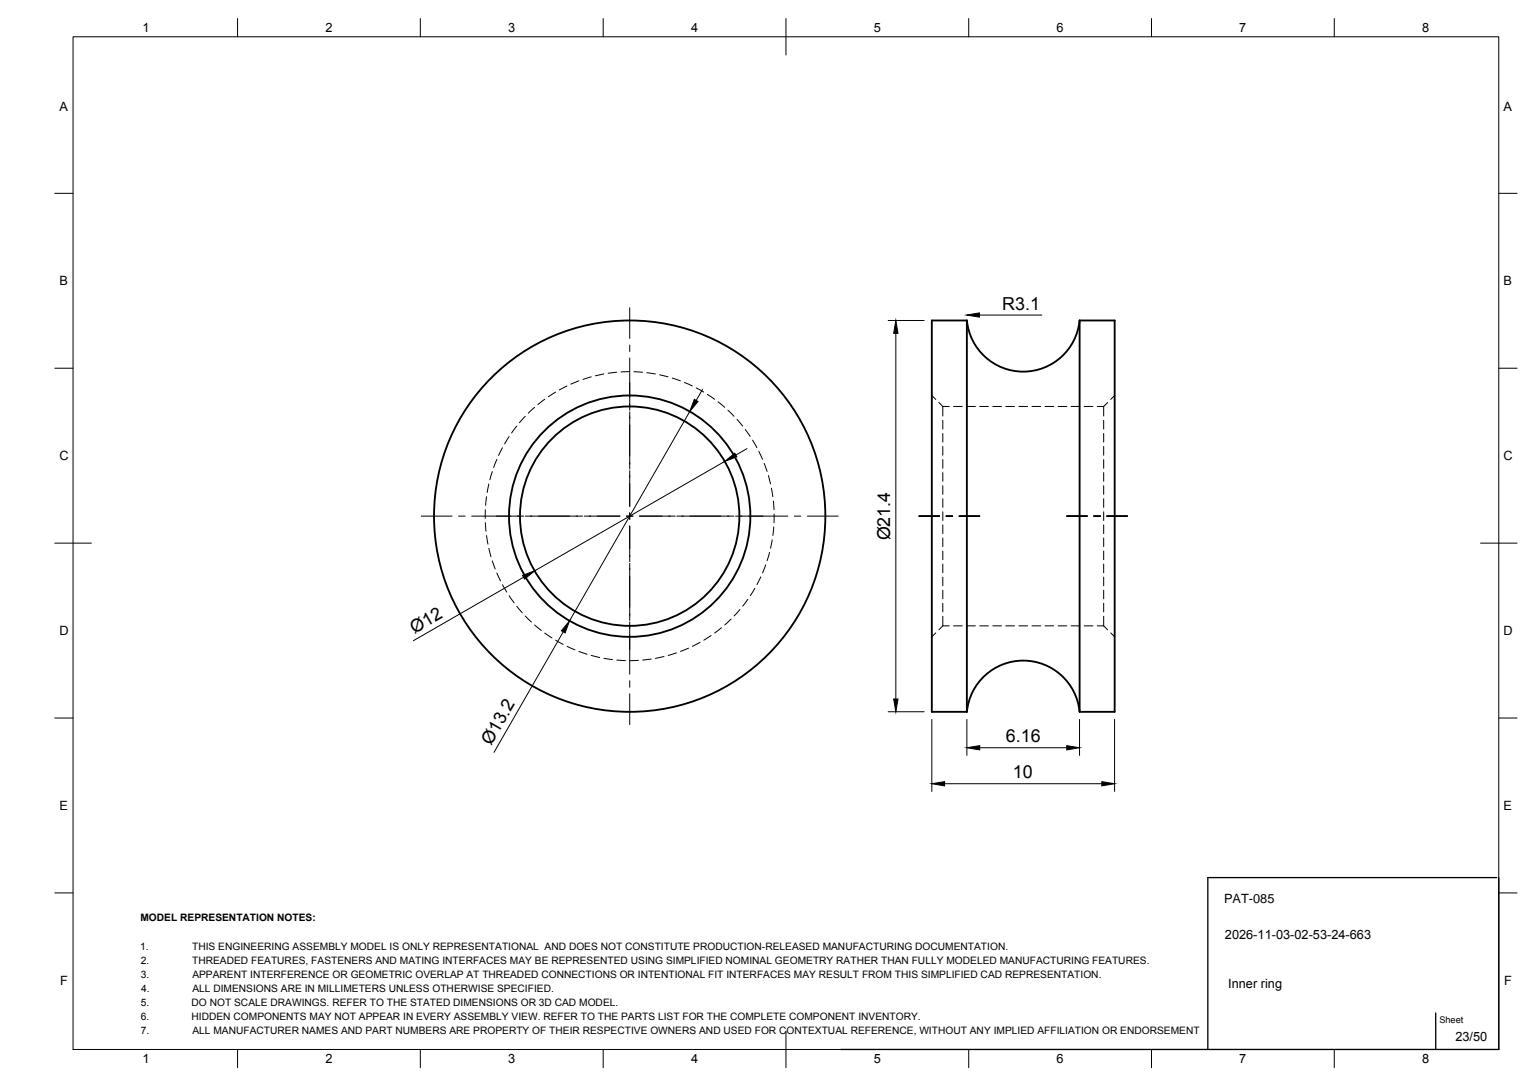
ISO-10303-21;
HEADER;
/* Generated by software containing ST-Developer
 * from STEP Tools, Inc. (www.steptools.com) 
 */

FILE_DESCRIPTION(
/* description */ ('Rack and pinion manual slide'),
/* implementation_level */ '2;1');

FILE_NAME(
/* name */ 'Inner ring.step',
/* time_stamp */ '2026-10-28T03:22:49-07:00',
/* author */ (''),
/* organization */ (''),
/* preprocessor_version */ 'ST-DEVELOPER v20.2',
/* originating_system */ 'Autodesk Translation Framework v15.17.0.0',
/* authorisation */ '');

FILE_SCHEMA (('AUTOMOTIVE_DESIGN { 1 0 10303 214 3 1 1 }'));
ENDSEC;

DATA;
#10=MECHANICAL_DESIGN_GEOMETRIC_PRESENTATION_REPRESENTATION('',(#751),#34851);
#603=TOROIDAL_SURFACE('',#14780,1.1,0.309556);
#620=CONICAL_SURFACE('',#14791,0.63,0.785398163397448);
#621=CONICAL_SURFACE('',#14798,0.63,0.785398163397448);
#659=SHAPE_REPRESENTATION_RELATIONSHIP('SRR','None',#35095,#705);
#705=ADVANCED_BREP_SHAPE_REPRESENTATION('',(#803),#34820);
#751=STYLED_ITEM('',(#35411),#803);
#803=MANIFOLD_SOLID_BREP('Body1',#13772);
#975=FACE_BOUND('',#2684,.T.);
#976=FACE_BOUND('',#2687,.T.);
#1218=PLANE('',#14793);
#1219=PLANE('',#14796);
#1798=FACE_OUTER_BOUND('',#2679,.T.);
#1799=FACE_OUTER_BOUND('',#2680,.T.);
#1800=FACE_OUTER_BOUND('',#2681,.T.);
#1801=FACE_OUTER_BOUND('',#2682,.T.);
#1802=FACE_OUTER_BOUND('',#2683,.T.);
#1803=FACE_OUTER_BOUND('',#2685,.T.);
#1804=FACE_OUTER_BOUND('',#2686,.T.);
#1805=FACE_OUTER_BOUND('',#2688,.T.);
#2679=EDGE_LOOP('',(#10490,#10491,#10492,#10493,#10494,#10495));
#2680=EDGE_LOOP('',(#10496,#10497,#10498,#10499,#10500));
#2681=EDGE_LOOP('',(#10501,#10502,#10503,#10504));
#2682=EDGE_LOOP('',(#10505,#10506,#10507,#10508));
#2683=EDGE_LOOP('',(#10509));
#2684=EDGE_LOOP('',(#10510));
#2685=EDGE_LOOP('',(#10511,#10512,#10513,#10514,#10515));
#2686=EDGE_LOOP('',(#10516));
#2687=EDGE_LOOP('',(#10517));
#2688=EDGE_LOOP('',(#10518,#10519,#10520,#10521));
#3675=LINE('',#20800,#4966);
#3676=LINE('',#20806,#4967);
#3677=LINE('',#20810,#4968);
#3678=LINE('',#20816,#4969);
#3679=LINE('',#20821,#4970);
#4966=VECTOR('',#16991,1.070235);
#4967=VECTOR('',#16998,0.6);
#4968=VECTOR('',#17003,0.63);
#4969=VECTOR('',#17012,1.070235);
#4970=VECTOR('',#17019,0.63);
#5981=CIRCLE('',#14781,1.070235);
#5982=CIRCLE('',#14782,1.070235);
#5983=CIRCLE('',#14783,0.309556);
#5984=CIRCLE('',#14784,1.070235);
#5985=CIRCLE('',#14785,1.070235);
#5986=CIRCLE('',#14787,1.070235);
#5987=CIRCLE('',#14789,0.6);
#5988=CIRCLE('',#14790,0.6);
#5989=CIRCLE('',#14792,0.66);
#5990=CIRCLE('',#14795,1.070235);
#5991=CIRCLE('',#14797,0.66);
#6641=VERTEX_POINT('',#20789);
#6642=VERTEX_POINT('',#20790);
#6643=VERTEX_POINT('',#20793);
#6644=VERTEX_POINT('',#20795);
#6645=VERTEX_POINT('',#20799);
#6646=VERTEX_POINT('',#20803);
#6647=VERTEX_POINT('',#20805);
#6648=VERTEX_POINT('',#20809);
#6649=VERTEX_POINT('',#20814);
#6650=VERTEX_POINT('',#20818);
#8057=EDGE_CURVE('',#6641,#6642,#5981,.T.);
#8058=EDGE_CURVE('',#6642,#6641,#5982,.T.);
#8059=EDGE_CURVE('',#6642,#6643,#5983,.T.);
#8060=EDGE_CURVE('',#6644,#6643,#5984,.T.);
#8061=EDGE_CURVE('',#6643,#6644,#5985,.T.);
#8062=EDGE_CURVE('',#6644,#6645,#3675,.T.);
#8063=EDGE_CURVE('',#6645,#6645,#5986,.T.);
#8064=EDGE_CURVE('',#6646,#6646,#5987,.T.);
#8065=EDGE_CURVE('',#6646,#6647,#3676,.T.);
#8066=EDGE_CURVE('',#6647,#6647,#5988,.T.);
#8067=EDGE_CURVE('',#6647,#6648,#3677,.T.);
#8068=EDGE_CURVE('',#6648,#6648,#5989,.T.);
#8069=EDGE_CURVE('',#6649,#6649,#5990,.T.);
#8070=EDGE_CURVE('',#6649,#6641,#3678,.T.);
#8071=EDGE_CURVE('',#6650,#6650,#5991,.T.);
#8072=EDGE_CURVE('',#6650,#6646,#3679,.T.);
#10490=ORIENTED_EDGE('',*,*,#8057,.F.);
#10491=ORIENTED_EDGE('',*,*,#8058,.F.);
#10492=ORIENTED_EDGE('',*,*,#8059,.T.);
#10493=ORIENTED_EDGE('',*,*,#8060,.F.);
#10494=ORIENTED_EDGE('',*,*,#8061,.F.);
#10495=ORIENTED_EDGE('',*,*,#8059,.F.);
#10496=ORIENTED_EDGE('',*,*,#8060,.T.);
#10497=ORIENTED_EDGE('',*,*,#8061,.T.);
#10498=ORIENTED_EDGE('',*,*,#8062,.T.);
#10499=ORIENTED_EDGE('',*,*,#8063,.T.);
#10500=ORIENTED_EDGE('',*,*,#8062,.F.);
#10501=ORIENTED_EDGE('',*,*,#8064,.T.);
#10502=ORIENTED_EDGE('',*,*,#8065,.T.);
#10503=ORIENTED_EDGE('',*,*,#8066,.F.);
#10504=ORIENTED_EDGE('',*,*,#8065,.F.);
#10505=ORIENTED_EDGE('',*,*,#8066,.T.);
#10506=ORIENTED_EDGE('',*,*,#8067,.T.);
#10507=ORIENTED_EDGE('',*,*,#8068,.F.);
#10508=ORIENTED_EDGE('',*,*,#8067,.F.);
#10509=ORIENTED_EDGE('',*,*,#8063,.F.);
#10510=ORIENTED_EDGE('',*,*,#8068,.T.);
#10511=ORIENTED_EDGE('',*,*,#8069,.F.);
#10512=ORIENTED_EDGE('',*,*,#8070,.T.);
#10513=ORIENTED_EDGE('',*,*,#8057,.T.);
#10514=ORIENTED_EDGE('',*,*,#8058,.T.);
#10515=ORIENTED_EDGE('',*,*,#8070,.F.);
#10516=ORIENTED_EDGE('',*,*,#8069,.T.);
#10517=ORIENTED_EDGE('',*,*,#8071,.F.);
#10518=ORIENTED_EDGE('',*,*,#8071,.T.);
#10519=ORIENTED_EDGE('',*,*,#8072,.T.);
#10520=ORIENTED_EDGE('',*,*,#8064,.F.);
#10521=ORIENTED_EDGE('',*,*,#8072,.F.);
#12928=CYLINDRICAL_SURFACE('',#14786,1.070235);
#12929=CYLINDRICAL_SURFACE('',#14788,0.6);
#12930=CYLINDRICAL_SURFACE('',#14794,1.070235);
#13276=ADVANCED_FACE('',(#1798),#603,.F.);
#13277=ADVANCED_FACE('',(#1799),#12928,.T.);
#13278=ADVANCED_FACE('',(#1800),#12929,.F.);
#13279=ADVANCED_FACE('',(#1801),#620,.F.);
#13280=ADVANCED_FACE('',(#1802,#975),#1218,.T.);
#13281=ADVANCED_FACE('',(#1803),#12930,.T.);
#13282=ADVANCED_FACE('',(#1804,#976),#1219,.T.);
#13283=ADVANCED_FACE('',(#1805),#621,.F.);
#13772=CLOSED_SHELL('',(#13276,#13277,#13278,#13279,#13280,#13281,#13282,
#13283));
#14779=AXIS2_PLACEMENT_3D('',#20787,#16975,#16976);
#14780=AXIS2_PLACEMENT_3D('',#20788,#16977,#16978);
#14781=AXIS2_PLACEMENT_3D('',#20791,#16979,#16980);
#14782=AXIS2_PLACEMENT_3D('',#20792,#16981,#16982);
#14783=AXIS2_PLACEMENT_3D('',#20794,#16983,#16984);
#14784=AXIS2_PLACEMENT_3D('',#20796,#16985,#16986);
#14785=AXIS2_PLACEMENT_3D('',#20797,#16987,#16988);
#14786=AXIS2_PLACEMENT_3D('',#20798,#16989,#16990);
#14787=AXIS2_PLACEMENT_3D('',#20801,#16992,#16993);
#14788=AXIS2_PLACEMENT_3D('',#20802,#16994,#16995);
#14789=AXIS2_PLACEMENT_3D('',#20804,#16996,#16997);
#14790=AXIS2_PLACEMENT_3D('',#20807,#16999,#17000);
#14791=AXIS2_PLACEMENT_3D('',#20808,#17001,#17002);
#14792=AXIS2_PLACEMENT_3D('',#20811,#17004,#17005);
#14793=AXIS2_PLACEMENT_3D('',#20812,#17006,#17007);
#14794=AXIS2_PLACEMENT_3D('',#20813,#17008,#17009);
#14795=AXIS2_PLACEMENT_3D('',#20815,#17010,#17011);
#14796=AXIS2_PLACEMENT_3D('',#20817,#17013,#17014);
#14797=AXIS2_PLACEMENT_3D('',#20819,#17015,#17016);
#14798=AXIS2_PLACEMENT_3D('',#20820,#17017,#17018);
#16975=DIRECTION('axis',(0.,0.,1.));
#16976=DIRECTION('refdir',(1.,0.,0.));
#16977=DIRECTION('center_axis',(0.,-1.,0.));
#16978=DIRECTION('ref_axis',(0.,0.,-1.));
#16979=DIRECTION('center_axis',(0.,-1.,0.));
#16980=DIRECTION('ref_axis',(1.,0.,0.));
#16981=DIRECTION('center_axis',(0.,-1.,0.));
#16982=DIRECTION('ref_axis',(1.,0.,0.));
#16983=DIRECTION('center_axis',(1.,0.,1.22464679914735E-16));
#16984=DIRECTION('ref_axis',(-1.22464679914735E-16,0.,1.));
#16985=DIRECTION('center_axis',(0.,1.,0.));
#16986=DIRECTION('ref_axis',(1.,0.,0.));
#16987=DIRECTION('center_axis',(0.,1.,0.));
#16988=DIRECTION('ref_axis',(1.,0.,0.));
#16989=DIRECTION('center_axis',(0.,-1.,0.));
#16990=DIRECTION('ref_axis',(1.,0.,0.));
#16991=DIRECTION('',(0.,1.,0.));
#16992=DIRECTION('center_axis',(0.,-1.,0.));
#16993=DIRECTION('ref_axis',(1.,0.,0.));
#16994=DIRECTION('center_axis',(0.,-1.,0.));
#16995=DIRECTION('ref_axis',(1.,0.,0.));
#16996=DIRECTION('center_axis',(0.,-1.,0.));
#16997=DIRECTION('ref_axis',(1.,0.,0.));
#16998=DIRECTION('',(0.,1.,0.));
#16999=DIRECTION('center_axis',(0.,-1.,0.));
#17000=DIRECTION('ref_axis',(1.,0.,0.));
#17001=DIRECTION('center_axis',(0.,1.,0.));
#17002=DIRECTION('ref_axis',(1.,0.,0.));
#17003=DIRECTION('',(-0.707106781186548,0.707106781186547,-8.65956056235493E-17));
#17004=DIRECTION('center_axis',(0.,-1.,0.));
#17005=DIRECTION('ref_axis',(1.,0.,0.));
#17006=DIRECTION('center_axis',(0.,1.,0.));
#17007=DIRECTION('ref_axis',(0.,0.,1.));
#17008=DIRECTION('center_axis',(0.,-1.,0.));
#17009=DIRECTION('ref_axis',(1.,0.,0.));
#17010=DIRECTION('center_axis',(0.,-1.,0.));
#17011=DIRECTION('ref_axis',(1.,0.,0.));
#17012=DIRECTION('',(0.,1.,0.));
#17013=DIRECTION('center_axis',(0.,-1.,0.));
#17014=DIRECTION('ref_axis',(0.,0.,-1.));
#17015=DIRECTION('center_axis',(0.,-1.,0.));
#17016=DIRECTION('ref_axis',(1.,0.,0.));
#17017=DIRECTION('center_axis',(0.,-1.,0.));
#17018=DIRECTION('ref_axis',(1.,0.,0.));
#17019=DIRECTION('',(0.707106781186548,0.707106781186547,8.65956056235493E-17));
#20787=CARTESIAN_POINT('',(0.,0.,0.));
#20788=CARTESIAN_POINT('Origin',(0.,0.,0.));
#20789=CARTESIAN_POINT('',(-1.070235,-0.308121667383195,-1.31065986708547E-16));
#20790=CARTESIAN_POINT('',(-1.31065986708547E-16,-0.308121667383195,1.070235));
#20791=CARTESIAN_POINT('Origin',(0.,-0.308121667383195,0.));
#20792=CARTESIAN_POINT('Origin',(0.,-0.308121667383195,0.));
#20793=CARTESIAN_POINT('',(-1.31065986708547E-16,0.308121667383195,1.070235));
#20794=CARTESIAN_POINT('Origin',(-1.34711147906209E-16,0.,1.1));
#20795=CARTESIAN_POINT('',(-1.070235,0.308121667383195,1.31065986708547E-16));
#20796=CARTESIAN_POINT('Origin',(0.,0.308121667383195,0.));
#20797=CARTESIAN_POINT('Origin',(0.,0.308121667383195,0.));
#20798=CARTESIAN_POINT('Origin',(0.,0.,0.));
#20799=CARTESIAN_POINT('',(-1.070235,0.5,-1.31065986708547E-16));
#20800=CARTESIAN_POINT('',(-1.070235,0.,-1.31065986708547E-16));
#20801=CARTESIAN_POINT('Origin',(0.,0.5,0.));
#20802=CARTESIAN_POINT('Origin',(0.,0.,0.));
#20803=CARTESIAN_POINT('',(-0.6,-0.44,-7.34788079488412E-17));
#20804=CARTESIAN_POINT('Origin',(0.,-0.44,0.));
#20805=CARTESIAN_POINT('',(-0.6,0.44,-7.34788079488412E-17));
#20806=CARTESIAN_POINT('',(-0.6,0.,-7.34788079488412E-17));
#20807=CARTESIAN_POINT('Origin',(0.,0.44,0.));
#20808=CARTESIAN_POINT('Origin',(0.,0.47,0.));
#20809=CARTESIAN_POINT('',(-0.66,0.5,-8.08266887437253E-17));
#20810=CARTESIAN_POINT('',(-0.63,0.47,-7.71527483462832E-17));
#20811=CARTESIAN_POINT('Origin',(0.,0.5,0.));
#20812=CARTESIAN_POINT('Origin',(1.070235,0.5,0.));
#20813=CARTESIAN_POINT('Origin',(0.,0.,0.));
#20814=CARTESIAN_POINT('',(-1.070235,-0.5,-1.31065986708547E-16));
#20815=CARTESIAN_POINT('Origin',(0.,-0.5,0.));
#20816=CARTESIAN_POINT('',(-1.070235,0.,-1.31065986708547E-16));
#20817=CARTESIAN_POINT('Origin',(0.66,-0.5,0.));
#20818=CARTESIAN_POINT('',(-0.66,-0.5,-8.08266887437253E-17));
#20819=CARTESIAN_POINT('Origin',(0.,-0.5,0.));
#20820=CARTESIAN_POINT('Origin',(0.,-0.47,0.));
#20821=CARTESIAN_POINT('',(-0.63,-0.47,-7.71527483462832E-17));
#34766=UNCERTAINTY_MEASURE_WITH_UNIT(LENGTH_MEASURE(0.001),#34852,
'DISTANCE_ACCURACY_VALUE',
'Maximum model space distance between geometric entities at asserted c
onnectivities');
#34797=UNCERTAINTY_MEASURE_WITH_UNIT(LENGTH_MEASURE(0.001),#34852,
'DISTANCE_ACCURACY_VALUE',
'Maximum model space distance between geometric entities at asserted c
onnectivities');
#34820=(
GEOMETRIC_REPRESENTATION_CONTEXT(3)
GLOBAL_UNCERTAINTY_ASSIGNED_CONTEXT((#34766))
GLOBAL_UNIT_ASSIGNED_CONTEXT((#34852,#34854,#34855))
REPRESENTATION_CONTEXT('','3D')
);
#34851=(
GEOMETRIC_REPRESENTATION_CONTEXT(3)
GLOBAL_UNCERTAINTY_ASSIGNED_CONTEXT((#34797))
GLOBAL_UNIT_ASSIGNED_CONTEXT((#34852,#34854,#34855))
REPRESENTATION_CONTEXT('','3D')
);
#34852=(
LENGTH_UNIT()
NAMED_UNIT(*)
SI_UNIT(.CENTI.,.METRE.)
);
#34854=(
NAMED_UNIT(*)
PLANE_ANGLE_UNIT()
SI_UNIT($,.RADIAN.)
);
#34855=(
NAMED_UNIT(*)
SI_UNIT($,.STERADIAN.)
SOLID_ANGLE_UNIT()
);
#34878=SHAPE_DEFINITION_REPRESENTATION(#34931,#35095);
#34931=PRODUCT_DEFINITION_SHAPE('',$,#35149);
#35095=SHAPE_REPRESENTATION('',(#14779),#34820);
#35126=PRODUCT_DEFINITION_CONTEXT('part definition',#35287,'design');
#35149=PRODUCT_DEFINITION('Inner ring','Inner ring',#35202,#35126);
#35202=PRODUCT_DEFINITION_FORMATION('',$,#35311);
#35287=APPLICATION_CONTEXT(
'Core Data for Automotive Mechanical Design Process');
#35288=PRODUCT_CONTEXT('part definition',#35287,'mechanical');
#35311=PRODUCT('Inner ring','Inner ring','Inner ring',(#35288));
#35405=COLOUR_RGB('Grey',0.48,0.52,0.57);
#35406=FILL_AREA_STYLE_COLOUR('',#35405);
#35407=FILL_AREA_STYLE('',(#35406));
#35408=SURFACE_STYLE_FILL_AREA(#35407);
#35409=SURFACE_SIDE_STYLE('',(#35408));
#35410=SURFACE_STYLE_USAGE(.BOTH.,#35409);
#35411=PRESENTATION_STYLE_ASSIGNMENT((#35410));
ENDSEC;
END-ISO-10303-21;
